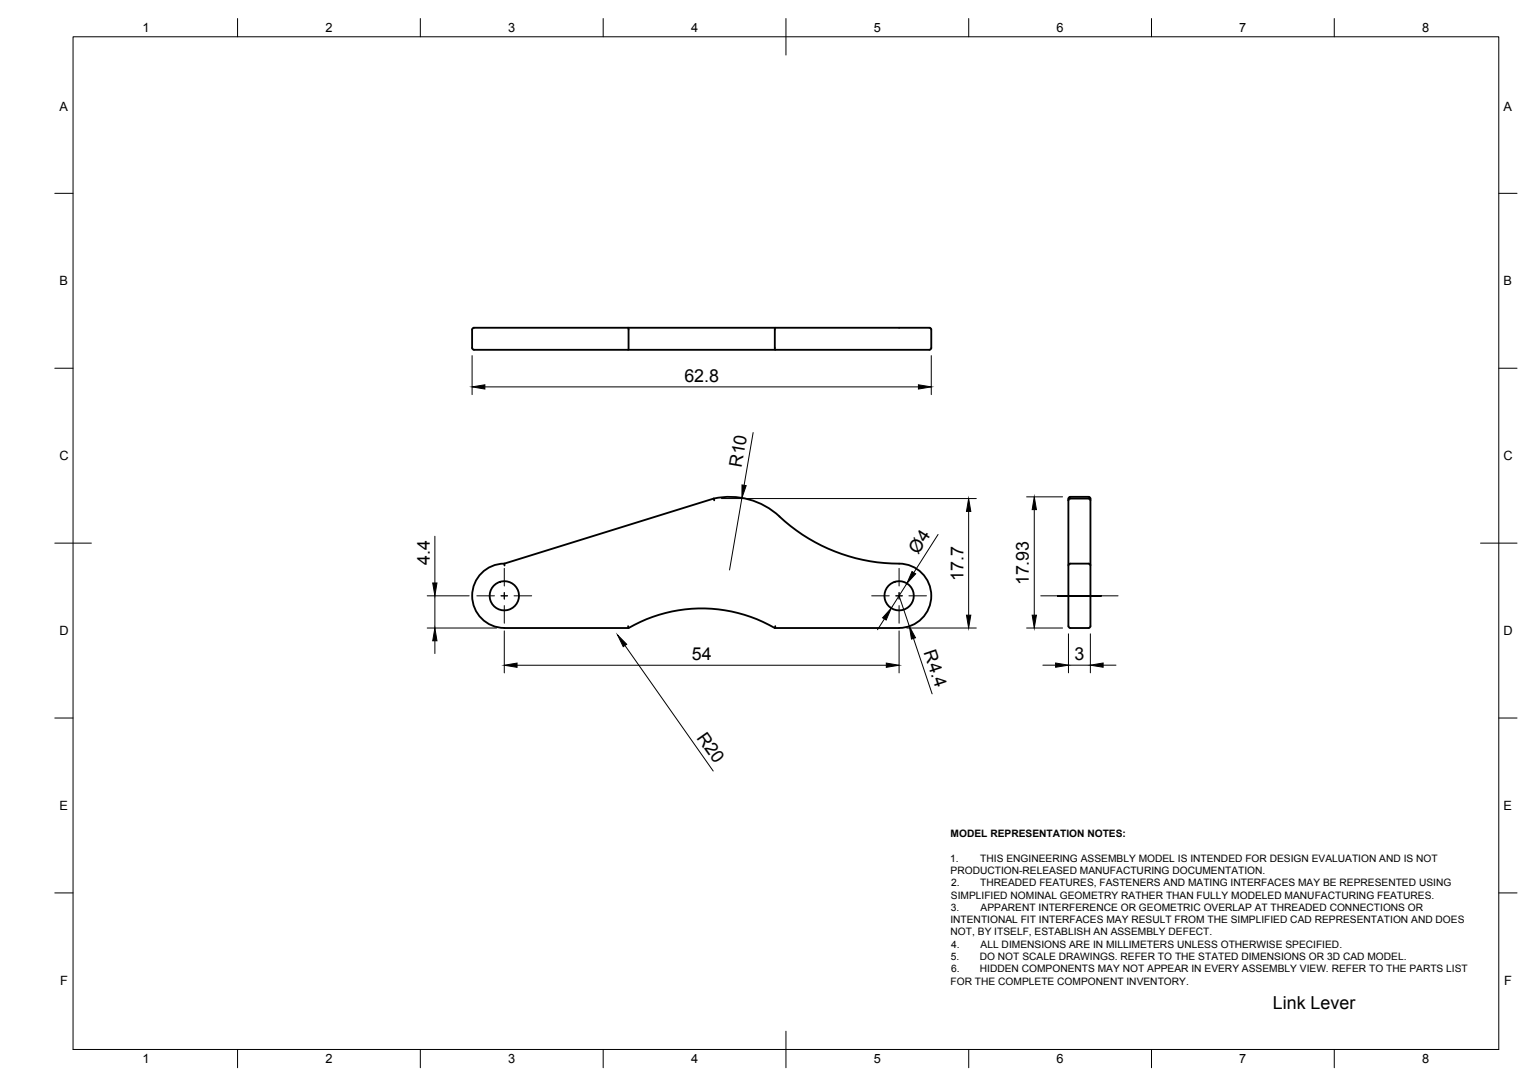
ISO-10303-21;
HEADER;
/* Generated by software containing ST-Developer
 * from STEP Tools, Inc. (www.steptools.com) 
 */

FILE_DESCRIPTION(
/* description */ ('STEP AP214'),
/* implementation_level */ '2;1');

FILE_NAME(
/* name */ 'Link Lever.step',
/* time_stamp */ '2026-10-06T11:11:25-07:00',
/* author */ (''),
/* organization */ (''),
/* preprocessor_version */ 'ST-DEVELOPER v20.2',
/* originating_system */ 'Autodesk Translation Framework v15.15.0.0',
/* authorisation */ '');

FILE_SCHEMA (('AUTOMOTIVE_DESIGN { 1 0 10303 214 3 1 1 }'));
ENDSEC;

DATA;
#10=MECHANICAL_DESIGN_GEOMETRIC_PRESENTATION_REPRESENTATION('',(#709),#47717);
#518=B_SPLINE_CURVE_WITH_KNOTS('',3,(#47531,#47532,#47533,#47534,#47535,
#47536,#47537,#47538,#47539,#47540,#47541,#47542,#47543,#47544),
 .UNSPECIFIED.,.F.,.F.,(4,2,2,2,2,2,4),(0.039886669715827,0.0401044661515991,
0.0495727843168759,0.0592161981418575,0.0692076983643014,0.0797697497054474,
0.0800012054326904),.UNSPECIFIED.);
#519=B_SPLINE_CURVE_WITH_KNOTS('',3,(#47547,#47548,#47549,#47550,#47551,
#47552,#47553,#47554,#47555,#47556,#47557,#47558),.UNSPECIFIED.,.F.,.F.,
(4,2,2,2,2,4),(-0.000230133150951674,0.,0.0101766413292995,0.0200160913840905,
0.0297402908990685,0.0394076883089345),.UNSPECIFIED.);
#520=B_SPLINE_CURVE_WITH_KNOTS('',3,(#47560,#47561,#47562,#47563,#47564,
#47565,#47566,#47567,#47568,#47569,#47570,#47571),.UNSPECIFIED.,.F.,.F.,
(4,2,2,2,2,4),(-0.0398866697156879,-0.0305471274410706,-0.0206752787312571,
-0.010434866365749,0.,0.000231445227518166),.UNSPECIFIED.);
#521=B_SPLINE_CURVE_WITH_KNOTS('',3,(#47573,#47574,#47575,#47576,#47577,
#47578,#47579,#47580,#47581,#47582,#47583,#47584,#47585,#47586,#47587,#47588,
#47589,#47590,#47591,#47592,#47593,#47594,#47595,#47596,#47597,#47598,#47599,
#47600),.UNSPECIFIED.,.F.,.F.,(4,3,3,3,3,3,3,3,3,4),(-1.09105494845026E-5,
3.84251023745443E-5,8.55160249623879E-5,0.000132661739759183,0.000179909175493616,
0.000186432057951685,0.00023702907904941,0.000287481797438324,0.000337436285325506,
0.000383774665387872),.UNSPECIFIED.);
#522=B_SPLINE_CURVE_WITH_KNOTS('',3,(#47606,#47607,#47608,#47609,#47610,
#47611,#47612,#47613,#47614,#47615,#47616,#47617),.UNSPECIFIED.,.F.,.F.,
(4,2,2,2,2,4),(-0.0790455097686946,-0.0788153766177156,-0.0686387352884633,
-0.0587992852337163,-0.0490750857187486,-0.0394076883088853),
 .UNSPECIFIED.);
#523=B_SPLINE_CURVE_WITH_KNOTS('',3,(#47618,#47619,#47620,#47621,#47622,
#47623,#47624,#47625,#47626,#47627,#47628,#47629,#47630,#47631,#47632,#47633,
#47634,#47635,#47636,#47637,#47638,#47639,#47640,#47641,#47642,#47643,#47644,
#47645),.UNSPECIFIED.,.F.,.F.,(4,3,3,3,3,3,3,3,3,4),(0.,4.94468472281981E-5,
9.92247531380756E-5,0.00014929675610942,0.000195377841020618,0.000238646755348352,
0.000281883277306065,0.00032509948720421,0.000368395674290727,0.000390755682041237),
 .UNSPECIFIED.);
#524=B_SPLINE_CURVE_WITH_KNOTS('',3,(#47652,#47653,#47654,#47655,#47656,
#47657,#47658,#47659,#47660,#47661,#47662,#47663),.UNSPECIFIED.,.F.,.F.,
(4,2,2,2,2,4),(-0.000231445227522379,0.,0.0104348663658747,0.0206752787314242,
0.0305471274412819,0.0398866697158144),.UNSPECIFIED.);
#525=B_SPLINE_CURVE_WITH_KNOTS('',3,(#47665,#47666,#47667,#47668,#47669,
#47670,#47671,#47672,#47673,#47674,#47675,#47676),.UNSPECIFIED.,.F.,.F.,
(4,2,2,2,2,4),(-0.0799975657698679,-0.0797661310415978,-0.0693317380416801,
-0.0590917902207848,-0.0492203893360867,-0.0398812707391191),
 .UNSPECIFIED.);
#660=TOROIDAL_SURFACE('',#9872,2.25,0.25);
#661=TOROIDAL_SURFACE('',#9876,4.15,0.25);
#662=TOROIDAL_SURFACE('',#9881,2.25,0.25);
#663=TOROIDAL_SURFACE('',#9885,4.15,0.25);
#664=TOROIDAL_SURFACE('',#9890,2.25,0.25);
#665=TOROIDAL_SURFACE('',#9894,2.25,0.25);
#666=TOROIDAL_SURFACE('',#9928,4.15,0.25);
#667=TOROIDAL_SURFACE('',#9929,20.25,0.25);
#668=TOROIDAL_SURFACE('',#9932,9.75,0.25);
#669=TOROIDAL_SURFACE('',#9934,24.25,0.25);
#670=TOROIDAL_SURFACE('',#9936,9.75,0.25);
#671=TOROIDAL_SURFACE('',#9938,4.15,0.25);
#672=TOROIDAL_SURFACE('',#9940,24.25,0.25);
#673=TOROIDAL_SURFACE('',#9942,20.25,0.25);
#685=SHAPE_REPRESENTATION_RELATIONSHIP('SRR','None',#47772,#697);
#697=ADVANCED_BREP_SHAPE_REPRESENTATION('',(#721),#47716);
#709=STYLED_ITEM('',(#47830),#721);
#721=MANIFOLD_SOLID_BREP('Body1',#8936);
#755=FACE_BOUND('',#3098,.T.);
#756=FACE_BOUND('',#3099,.T.);
#757=FACE_BOUND('',#3101,.T.);
#758=FACE_BOUND('',#3102,.T.);
#878=PLANE('',#9901);
#879=PLANE('',#9906);
#880=PLANE('',#9911);
#881=PLANE('',#9915);
#882=PLANE('',#9919);
#1348=LINE('',#47457,#1835);
#1349=LINE('',#47459,#1836);
#1350=LINE('',#47461,#1837);
#1351=LINE('',#47462,#1838);
#1352=LINE('',#47469,#1839);
#1353=LINE('',#47473,#1840);
#1354=LINE('',#47476,#1841);
#1355=LINE('',#47481,#1842);
#1356=LINE('',#47487,#1843);
#1357=LINE('',#47490,#1844);
#1358=LINE('',#47494,#1845);
#1359=LINE('',#47495,#1846);
#1360=LINE('',#47496,#1847);
#1361=LINE('',#47500,#1848);
#1362=LINE('',#47506,#1849);
#1363=LINE('',#47507,#1850);
#1364=LINE('',#47508,#1851);
#1365=LINE('',#47512,#1852);
#1366=LINE('',#47518,#1853);
#1367=LINE('',#47519,#1854);
#1368=LINE('',#47520,#1855);
#1369=LINE('',#47524,#1856);
#1835=VECTOR('',#12079,1.99999999999999);
#1836=VECTOR('',#12082,2.);
#1837=VECTOR('',#12085,1000.);
#1838=VECTOR('',#12086,1000.);
#1839=VECTOR('',#12093,1000.);
#1840=VECTOR('',#12096,1000.);
#1841=VECTOR('',#12099,1000.);
#1842=VECTOR('',#12104,1000.);
#1843=VECTOR('',#12109,1000.);
#1844=VECTOR('',#12112,1000.);
#1845=VECTOR('',#12115,1000.);
#1846=VECTOR('',#12116,1000.);
#1847=VECTOR('',#12117,1000.);
#1848=VECTOR('',#12120,1000.);
#1849=VECTOR('',#12127,1000.);
#1850=VECTOR('',#12128,1000.);
#1851=VECTOR('',#12129,1000.);
#1852=VECTOR('',#12132,1000.);
#1853=VECTOR('',#12139,1000.);
#1854=VECTOR('',#12140,1000.);
#1855=VECTOR('',#12141,1000.);
#1856=VECTOR('',#12144,1000.);
#2050=CYLINDRICAL_SURFACE('',#9898,1.99999999999999);
#2051=CYLINDRICAL_SURFACE('',#9899,2.);
#2052=CYLINDRICAL_SURFACE('',#9900,4.4);
#2053=CYLINDRICAL_SURFACE('',#9912,20.);
#2054=CYLINDRICAL_SURFACE('',#9916,4.4);
#2055=CYLINDRICAL_SURFACE('',#9920,9.99999999999999);
#2056=CYLINDRICAL_SURFACE('',#9923,24.);
#2057=CYLINDRICAL_SURFACE('',#9926,0.25);
#2058=CYLINDRICAL_SURFACE('',#9930,0.250000000000004);
#2059=CYLINDRICAL_SURFACE('',#9931,0.25);
#2060=CYLINDRICAL_SURFACE('',#9935,0.250000000000004);
#2061=CYLINDRICAL_SURFACE('',#9941,0.25);
#2062=CYLINDRICAL_SURFACE('',#9943,0.25);
#2543=FACE_OUTER_BOUND('',#3088,.T.);
#2544=FACE_OUTER_BOUND('',#3089,.T.);
#2545=FACE_OUTER_BOUND('',#3090,.T.);
#2546=FACE_OUTER_BOUND('',#3091,.T.);
#2547=FACE_OUTER_BOUND('',#3092,.T.);
#2548=FACE_OUTER_BOUND('',#3093,.T.);
#2549=FACE_OUTER_BOUND('',#3094,.T.);
#2550=FACE_OUTER_BOUND('',#3095,.T.);
#2551=FACE_OUTER_BOUND('',#3096,.T.);
#2552=FACE_OUTER_BOUND('',#3097,.T.);
#2553=FACE_OUTER_BOUND('',#3100,.T.);
#2554=FACE_OUTER_BOUND('',#3103,.T.);
#2555=FACE_OUTER_BOUND('',#3104,.T.);
#2556=FACE_OUTER_BOUND('',#3105,.T.);
#2557=FACE_OUTER_BOUND('',#3106,.T.);
#2558=FACE_OUTER_BOUND('',#3107,.T.);
#2559=FACE_OUTER_BOUND('',#3108,.T.);
#2560=FACE_OUTER_BOUND('',#3109,.T.);
#2561=FACE_OUTER_BOUND('',#3110,.T.);
#2562=FACE_OUTER_BOUND('',#3111,.T.);
#2563=FACE_OUTER_BOUND('',#3112,.T.);
#2564=FACE_OUTER_BOUND('',#3113,.T.);
#2565=FACE_OUTER_BOUND('',#3114,.T.);
#2566=FACE_OUTER_BOUND('',#3115,.T.);
#2567=FACE_OUTER_BOUND('',#3116,.T.);
#2568=FACE_OUTER_BOUND('',#3117,.T.);
#2569=FACE_OUTER_BOUND('',#3118,.T.);
#2570=FACE_OUTER_BOUND('',#3119,.T.);
#2571=FACE_OUTER_BOUND('',#3120,.T.);
#2572=FACE_OUTER_BOUND('',#3121,.T.);
#2573=FACE_OUTER_BOUND('',#3122,.T.);
#2574=FACE_OUTER_BOUND('',#3123,.T.);
#3088=EDGE_LOOP('',(#8263,#8264,#8265,#8266));
#3089=EDGE_LOOP('',(#8267,#8268,#8269,#8270));
#3090=EDGE_LOOP('',(#8271,#8272,#8273,#8274));
#3091=EDGE_LOOP('',(#8275,#8276,#8277,#8278));
#3092=EDGE_LOOP('',(#8279,#8280,#8281,#8282));
#3093=EDGE_LOOP('',(#8283,#8284,#8285,#8286));
#3094=EDGE_LOOP('',(#8287,#8288,#8289,#8290));
#3095=EDGE_LOOP('',(#8291,#8292,#8293,#8294));
#3096=EDGE_LOOP('',(#8295,#8296,#8297,#8298));
#3097=EDGE_LOOP('',(#8299,#8300,#8301,#8302,#8303,#8304,#8305,#8306));
#3098=EDGE_LOOP('',(#8307));
#3099=EDGE_LOOP('',(#8308));
#3100=EDGE_LOOP('',(#8309,#8310,#8311,#8312,#8313,#8314,#8315,#8316));
#3101=EDGE_LOOP('',(#8317));
#3102=EDGE_LOOP('',(#8318));
#3103=EDGE_LOOP('',(#8319,#8320,#8321,#8322));
#3104=EDGE_LOOP('',(#8323,#8324,#8325,#8326));
#3105=EDGE_LOOP('',(#8327,#8328,#8329,#8330));
#3106=EDGE_LOOP('',(#8331,#8332,#8333,#8334));
#3107=EDGE_LOOP('',(#8335,#8336,#8337,#8338));
#3108=EDGE_LOOP('',(#8339,#8340,#8341,#8342));
#3109=EDGE_LOOP('',(#8343,#8344,#8345,#8346));
#3110=EDGE_LOOP('',(#8347,#8348,#8349,#8350));
#3111=EDGE_LOOP('',(#8351,#8352,#8353,#8354));
#3112=EDGE_LOOP('',(#8355,#8356,#8357,#8358));
#3113=EDGE_LOOP('',(#8359,#8360,#8361,#8362));
#3114=EDGE_LOOP('',(#8363,#8364,#8365,#8366));
#3115=EDGE_LOOP('',(#8367,#8368,#8369,#8370));
#3116=EDGE_LOOP('',(#8371,#8372,#8373,#8374));
#3117=EDGE_LOOP('',(#8375,#8376,#8377,#8378));
#3118=EDGE_LOOP('',(#8379,#8380,#8381,#8382));
#3119=EDGE_LOOP('',(#8383,#8384,#8385,#8386));
#3120=EDGE_LOOP('',(#8387,#8388,#8389,#8390));
#3121=EDGE_LOOP('',(#8391,#8392,#8393,#8394));
#3122=EDGE_LOOP('',(#8395,#8396,#8397,#8398));
#3123=EDGE_LOOP('',(#8399,#8400,#8401,#8402));
#3492=CIRCLE('',#9873,2.);
#3493=CIRCLE('',#9874,0.25);
#3494=CIRCLE('',#9875,2.25);
#3495=CIRCLE('',#9877,4.4);
#3496=CIRCLE('',#9878,0.25);
#3497=CIRCLE('',#9879,4.15);
#3498=CIRCLE('',#9880,0.25);
#3499=CIRCLE('',#9882,1.99999999999999);
#3500=CIRCLE('',#9883,0.25);
#3501=CIRCLE('',#9884,2.24999999999999);
#3502=CIRCLE('',#9886,4.15);
#3503=CIRCLE('',#9887,0.25);
#3504=CIRCLE('',#9888,4.4);
#3505=CIRCLE('',#9889,0.25);
#3506=CIRCLE('',#9891,2.25);
#3507=CIRCLE('',#9892,0.25);
#3508=CIRCLE('',#9893,2.);
#3509=CIRCLE('',#9895,2.25);
#3510=CIRCLE('',#9896,0.25);
#3511=CIRCLE('',#9897,2.00000000000001);
#3512=CIRCLE('',#9902,9.75);
#3513=CIRCLE('',#9903,24.25);
#3514=CIRCLE('',#9904,20.25);
#3515=CIRCLE('',#9905,4.15);
#3516=CIRCLE('',#9907,20.25);
#3517=CIRCLE('',#9908,24.25);
#3518=CIRCLE('',#9909,9.74999999999999);
#3519=CIRCLE('',#9910,4.15);
#3520=CIRCLE('',#9913,20.);
#3521=CIRCLE('',#9914,20.);
#3522=CIRCLE('',#9917,4.4);
#3523=CIRCLE('',#9918,4.4);
#3524=CIRCLE('',#9921,9.99999999999999);
#3525=CIRCLE('',#9922,9.99999999999999);
#3526=CIRCLE('',#9924,24.);
#3527=CIRCLE('',#9925,24.);
#3528=CIRCLE('',#9927,0.25);
#3529=CIRCLE('',#9933,0.249999999999998);
#3530=CIRCLE('',#9937,0.249999999999998);
#3531=CIRCLE('',#9939,0.25);
#4349=VERTEX_POINT('',#47415);
#4350=VERTEX_POINT('',#47417);
#4351=VERTEX_POINT('',#47421);
#4352=VERTEX_POINT('',#47422);
#4353=VERTEX_POINT('',#47424);
#4354=VERTEX_POINT('',#47426);
#4355=VERTEX_POINT('',#47430);
#4356=VERTEX_POINT('',#47432);
#4357=VERTEX_POINT('',#47436);
#4358=VERTEX_POINT('',#47437);
#4359=VERTEX_POINT('',#47439);
#4360=VERTEX_POINT('',#47441);
#4361=VERTEX_POINT('',#47445);
#4362=VERTEX_POINT('',#47447);
#4363=VERTEX_POINT('',#47451);
#4364=VERTEX_POINT('',#47453);
#4365=VERTEX_POINT('',#47464);
#4366=VERTEX_POINT('',#47465);
#4367=VERTEX_POINT('',#47468);
#4368=VERTEX_POINT('',#47470);
#4369=VERTEX_POINT('',#47472);
#4370=VERTEX_POINT('',#47474);
#4371=VERTEX_POINT('',#47478);
#4372=VERTEX_POINT('',#47479);
#4373=VERTEX_POINT('',#47482);
#4374=VERTEX_POINT('',#47484);
#4375=VERTEX_POINT('',#47486);
#4376=VERTEX_POINT('',#47488);
#4377=VERTEX_POINT('',#47492);
#4378=VERTEX_POINT('',#47493);
#4379=VERTEX_POINT('',#47498);
#4380=VERTEX_POINT('',#47499);
#4381=VERTEX_POINT('',#47504);
#4382=VERTEX_POINT('',#47505);
#4383=VERTEX_POINT('',#47510);
#4384=VERTEX_POINT('',#47511);
#4385=VERTEX_POINT('',#47516);
#4386=VERTEX_POINT('',#47517);
#4387=VERTEX_POINT('',#47522);
#4388=VERTEX_POINT('',#47523);
#5657=EDGE_CURVE('',#4349,#4349,#3492,.T.);
#5658=EDGE_CURVE('',#4349,#4350,#3493,.T.);
#5659=EDGE_CURVE('',#4350,#4350,#3494,.T.);
#5660=EDGE_CURVE('',#4351,#4352,#3495,.T.);
#5661=EDGE_CURVE('',#4351,#4353,#3496,.T.);
#5662=EDGE_CURVE('',#4354,#4353,#3497,.T.);
#5663=EDGE_CURVE('',#4352,#4354,#3498,.T.);
#5664=EDGE_CURVE('',#4355,#4355,#3499,.T.);
#5665=EDGE_CURVE('',#4355,#4356,#3500,.T.);
#5666=EDGE_CURVE('',#4356,#4356,#3501,.T.);
#5667=EDGE_CURVE('',#4357,#4358,#3502,.T.);
#5668=EDGE_CURVE('',#4359,#4357,#3503,.T.);
#5669=EDGE_CURVE('',#4360,#4359,#3504,.T.);
#5670=EDGE_CURVE('',#4360,#4358,#3505,.T.);
#5671=EDGE_CURVE('',#4361,#4361,#3506,.T.);
#5672=EDGE_CURVE('',#4361,#4362,#3507,.T.);
#5673=EDGE_CURVE('',#4362,#4362,#3508,.T.);
#5674=EDGE_CURVE('',#4363,#4363,#3509,.T.);
#5675=EDGE_CURVE('',#4363,#4364,#3510,.T.);
#5676=EDGE_CURVE('',#4364,#4364,#3511,.T.);
#5677=EDGE_CURVE('',#4364,#4355,#1348,.T.);
#5678=EDGE_CURVE('',#4362,#4349,#1349,.T.);
#5679=EDGE_CURVE('',#4359,#4351,#1350,.T.);
#5680=EDGE_CURVE('',#4360,#4352,#1351,.T.);
#5681=EDGE_CURVE('',#4365,#4366,#3512,.T.);
#5682=EDGE_CURVE('',#4366,#4357,#3513,.T.);
#5683=EDGE_CURVE('',#4358,#4367,#1352,.T.);
#5684=EDGE_CURVE('',#4367,#4368,#3514,.T.);
#5685=EDGE_CURVE('',#4368,#4369,#1353,.T.);
#5686=EDGE_CURVE('',#4369,#4370,#3515,.T.);
#5687=EDGE_CURVE('',#4370,#4365,#1354,.T.);
#5688=EDGE_CURVE('',#4371,#4372,#3516,.T.);
#5689=EDGE_CURVE('',#4372,#4354,#1355,.T.);
#5690=EDGE_CURVE('',#4353,#4373,#3517,.T.);
#5691=EDGE_CURVE('',#4373,#4374,#3518,.T.);
#5692=EDGE_CURVE('',#4374,#4375,#1356,.T.);
#5693=EDGE_CURVE('',#4375,#4376,#3519,.T.);
#5694=EDGE_CURVE('',#4376,#4371,#1357,.T.);
#5695=EDGE_CURVE('',#4377,#4378,#1358,.T.);
#5696=EDGE_CURVE('',#4377,#4360,#1359,.T.);
#5697=EDGE_CURVE('',#4352,#4378,#1360,.T.);
#5698=EDGE_CURVE('',#4379,#4380,#1361,.T.);
#5699=EDGE_CURVE('',#4379,#4377,#3520,.T.);
#5700=EDGE_CURVE('',#4378,#4380,#3521,.T.);
#5701=EDGE_CURVE('',#4381,#4382,#1362,.T.);
#5702=EDGE_CURVE('',#4381,#4379,#1363,.T.);
#5703=EDGE_CURVE('',#4380,#4382,#1364,.T.);
#5704=EDGE_CURVE('',#4383,#4384,#1365,.T.);
#5705=EDGE_CURVE('',#4383,#4381,#3522,.T.);
#5706=EDGE_CURVE('',#4382,#4384,#3523,.T.);
#5707=EDGE_CURVE('',#4385,#4386,#1366,.T.);
#5708=EDGE_CURVE('',#4385,#4383,#1367,.T.);
#5709=EDGE_CURVE('',#4384,#4386,#1368,.T.);
#5710=EDGE_CURVE('',#4387,#4388,#1369,.T.);
#5711=EDGE_CURVE('',#4387,#4385,#3524,.T.);
#5712=EDGE_CURVE('',#4386,#4388,#3525,.T.);
#5713=EDGE_CURVE('',#4359,#4387,#3526,.T.);
#5714=EDGE_CURVE('',#4388,#4351,#3527,.T.);
#5715=EDGE_CURVE('',#4379,#4368,#518,.T.);
#5716=EDGE_CURVE('',#4369,#4381,#3528,.T.);
#5717=EDGE_CURVE('',#4370,#4383,#519,.T.);
#5718=EDGE_CURVE('',#4377,#4367,#520,.T.);
#5719=EDGE_CURVE('',#4365,#4385,#521,.T.);
#5720=EDGE_CURVE('',#4366,#4387,#3529,.T.);
#5721=EDGE_CURVE('',#4375,#4384,#522,.T.);
#5722=EDGE_CURVE('',#4386,#4374,#523,.T.);
#5723=EDGE_CURVE('',#4388,#4373,#3530,.T.);
#5724=EDGE_CURVE('',#4376,#4382,#3531,.T.);
#5725=EDGE_CURVE('',#4371,#4380,#524,.T.);
#5726=EDGE_CURVE('',#4372,#4378,#525,.T.);
#8263=ORIENTED_EDGE('',*,*,#5657,.F.);
#8264=ORIENTED_EDGE('',*,*,#5658,.T.);
#8265=ORIENTED_EDGE('',*,*,#5659,.F.);
#8266=ORIENTED_EDGE('',*,*,#5658,.F.);
#8267=ORIENTED_EDGE('',*,*,#5660,.F.);
#8268=ORIENTED_EDGE('',*,*,#5661,.T.);
#8269=ORIENTED_EDGE('',*,*,#5662,.F.);
#8270=ORIENTED_EDGE('',*,*,#5663,.F.);
#8271=ORIENTED_EDGE('',*,*,#5664,.F.);
#8272=ORIENTED_EDGE('',*,*,#5665,.T.);
#8273=ORIENTED_EDGE('',*,*,#5666,.F.);
#8274=ORIENTED_EDGE('',*,*,#5665,.F.);
#8275=ORIENTED_EDGE('',*,*,#5667,.F.);
#8276=ORIENTED_EDGE('',*,*,#5668,.F.);
#8277=ORIENTED_EDGE('',*,*,#5669,.F.);
#8278=ORIENTED_EDGE('',*,*,#5670,.T.);
#8279=ORIENTED_EDGE('',*,*,#5671,.F.);
#8280=ORIENTED_EDGE('',*,*,#5672,.T.);
#8281=ORIENTED_EDGE('',*,*,#5673,.F.);
#8282=ORIENTED_EDGE('',*,*,#5672,.F.);
#8283=ORIENTED_EDGE('',*,*,#5674,.F.);
#8284=ORIENTED_EDGE('',*,*,#5675,.T.);
#8285=ORIENTED_EDGE('',*,*,#5676,.F.);
#8286=ORIENTED_EDGE('',*,*,#5675,.F.);
#8287=ORIENTED_EDGE('',*,*,#5676,.T.);
#8288=ORIENTED_EDGE('',*,*,#5677,.T.);
#8289=ORIENTED_EDGE('',*,*,#5664,.T.);
#8290=ORIENTED_EDGE('',*,*,#5677,.F.);
#8291=ORIENTED_EDGE('',*,*,#5673,.T.);
#8292=ORIENTED_EDGE('',*,*,#5678,.T.);
#8293=ORIENTED_EDGE('',*,*,#5657,.T.);
#8294=ORIENTED_EDGE('',*,*,#5678,.F.);
#8295=ORIENTED_EDGE('',*,*,#5669,.T.);
#8296=ORIENTED_EDGE('',*,*,#5679,.T.);
#8297=ORIENTED_EDGE('',*,*,#5660,.T.);
#8298=ORIENTED_EDGE('',*,*,#5680,.F.);
#8299=ORIENTED_EDGE('',*,*,#5681,.T.);
#8300=ORIENTED_EDGE('',*,*,#5682,.T.);
#8301=ORIENTED_EDGE('',*,*,#5667,.T.);
#8302=ORIENTED_EDGE('',*,*,#5683,.T.);
#8303=ORIENTED_EDGE('',*,*,#5684,.T.);
#8304=ORIENTED_EDGE('',*,*,#5685,.T.);
#8305=ORIENTED_EDGE('',*,*,#5686,.T.);
#8306=ORIENTED_EDGE('',*,*,#5687,.T.);
#8307=ORIENTED_EDGE('',*,*,#5674,.T.);
#8308=ORIENTED_EDGE('',*,*,#5671,.T.);
#8309=ORIENTED_EDGE('',*,*,#5688,.T.);
#8310=ORIENTED_EDGE('',*,*,#5689,.T.);
#8311=ORIENTED_EDGE('',*,*,#5662,.T.);
#8312=ORIENTED_EDGE('',*,*,#5690,.T.);
#8313=ORIENTED_EDGE('',*,*,#5691,.T.);
#8314=ORIENTED_EDGE('',*,*,#5692,.T.);
#8315=ORIENTED_EDGE('',*,*,#5693,.T.);
#8316=ORIENTED_EDGE('',*,*,#5694,.T.);
#8317=ORIENTED_EDGE('',*,*,#5659,.T.);
#8318=ORIENTED_EDGE('',*,*,#5666,.T.);
#8319=ORIENTED_EDGE('',*,*,#5695,.F.);
#8320=ORIENTED_EDGE('',*,*,#5696,.T.);
#8321=ORIENTED_EDGE('',*,*,#5680,.T.);
#8322=ORIENTED_EDGE('',*,*,#5697,.T.);
#8323=ORIENTED_EDGE('',*,*,#5698,.F.);
#8324=ORIENTED_EDGE('',*,*,#5699,.T.);
#8325=ORIENTED_EDGE('',*,*,#5695,.T.);
#8326=ORIENTED_EDGE('',*,*,#5700,.T.);
#8327=ORIENTED_EDGE('',*,*,#5701,.F.);
#8328=ORIENTED_EDGE('',*,*,#5702,.T.);
#8329=ORIENTED_EDGE('',*,*,#5698,.T.);
#8330=ORIENTED_EDGE('',*,*,#5703,.T.);
#8331=ORIENTED_EDGE('',*,*,#5704,.F.);
#8332=ORIENTED_EDGE('',*,*,#5705,.T.);
#8333=ORIENTED_EDGE('',*,*,#5701,.T.);
#8334=ORIENTED_EDGE('',*,*,#5706,.T.);
#8335=ORIENTED_EDGE('',*,*,#5707,.F.);
#8336=ORIENTED_EDGE('',*,*,#5708,.T.);
#8337=ORIENTED_EDGE('',*,*,#5704,.T.);
#8338=ORIENTED_EDGE('',*,*,#5709,.T.);
#8339=ORIENTED_EDGE('',*,*,#5710,.F.);
#8340=ORIENTED_EDGE('',*,*,#5711,.T.);
#8341=ORIENTED_EDGE('',*,*,#5707,.T.);
#8342=ORIENTED_EDGE('',*,*,#5712,.T.);
#8343=ORIENTED_EDGE('',*,*,#5679,.F.);
#8344=ORIENTED_EDGE('',*,*,#5713,.T.);
#8345=ORIENTED_EDGE('',*,*,#5710,.T.);
#8346=ORIENTED_EDGE('',*,*,#5714,.T.);
#8347=ORIENTED_EDGE('',*,*,#5715,.F.);
#8348=ORIENTED_EDGE('',*,*,#5702,.F.);
#8349=ORIENTED_EDGE('',*,*,#5716,.F.);
#8350=ORIENTED_EDGE('',*,*,#5685,.F.);
#8351=ORIENTED_EDGE('',*,*,#5716,.T.);
#8352=ORIENTED_EDGE('',*,*,#5705,.F.);
#8353=ORIENTED_EDGE('',*,*,#5717,.F.);
#8354=ORIENTED_EDGE('',*,*,#5686,.F.);
#8355=ORIENTED_EDGE('',*,*,#5715,.T.);
#8356=ORIENTED_EDGE('',*,*,#5684,.F.);
#8357=ORIENTED_EDGE('',*,*,#5718,.F.);
#8358=ORIENTED_EDGE('',*,*,#5699,.F.);
#8359=ORIENTED_EDGE('',*,*,#5717,.T.);
#8360=ORIENTED_EDGE('',*,*,#5708,.F.);
#8361=ORIENTED_EDGE('',*,*,#5719,.F.);
#8362=ORIENTED_EDGE('',*,*,#5687,.F.);
#8363=ORIENTED_EDGE('',*,*,#5718,.T.);
#8364=ORIENTED_EDGE('',*,*,#5683,.F.);
#8365=ORIENTED_EDGE('',*,*,#5670,.F.);
#8366=ORIENTED_EDGE('',*,*,#5696,.F.);
#8367=ORIENTED_EDGE('',*,*,#5719,.T.);
#8368=ORIENTED_EDGE('',*,*,#5711,.F.);
#8369=ORIENTED_EDGE('',*,*,#5720,.F.);
#8370=ORIENTED_EDGE('',*,*,#5681,.F.);
#8371=ORIENTED_EDGE('',*,*,#5720,.T.);
#8372=ORIENTED_EDGE('',*,*,#5713,.F.);
#8373=ORIENTED_EDGE('',*,*,#5668,.T.);
#8374=ORIENTED_EDGE('',*,*,#5682,.F.);
#8375=ORIENTED_EDGE('',*,*,#5721,.F.);
#8376=ORIENTED_EDGE('',*,*,#5692,.F.);
#8377=ORIENTED_EDGE('',*,*,#5722,.F.);
#8378=ORIENTED_EDGE('',*,*,#5709,.F.);
#8379=ORIENTED_EDGE('',*,*,#5722,.T.);
#8380=ORIENTED_EDGE('',*,*,#5691,.F.);
#8381=ORIENTED_EDGE('',*,*,#5723,.F.);
#8382=ORIENTED_EDGE('',*,*,#5712,.F.);
#8383=ORIENTED_EDGE('',*,*,#5721,.T.);
#8384=ORIENTED_EDGE('',*,*,#5706,.F.);
#8385=ORIENTED_EDGE('',*,*,#5724,.F.);
#8386=ORIENTED_EDGE('',*,*,#5693,.F.);
#8387=ORIENTED_EDGE('',*,*,#5723,.T.);
#8388=ORIENTED_EDGE('',*,*,#5690,.F.);
#8389=ORIENTED_EDGE('',*,*,#5661,.F.);
#8390=ORIENTED_EDGE('',*,*,#5714,.F.);
#8391=ORIENTED_EDGE('',*,*,#5724,.T.);
#8392=ORIENTED_EDGE('',*,*,#5703,.F.);
#8393=ORIENTED_EDGE('',*,*,#5725,.F.);
#8394=ORIENTED_EDGE('',*,*,#5694,.F.);
#8395=ORIENTED_EDGE('',*,*,#5725,.T.);
#8396=ORIENTED_EDGE('',*,*,#5700,.F.);
#8397=ORIENTED_EDGE('',*,*,#5726,.F.);
#8398=ORIENTED_EDGE('',*,*,#5688,.F.);
#8399=ORIENTED_EDGE('',*,*,#5663,.T.);
#8400=ORIENTED_EDGE('',*,*,#5689,.F.);
#8401=ORIENTED_EDGE('',*,*,#5726,.T.);
#8402=ORIENTED_EDGE('',*,*,#5697,.F.);
#8893=ADVANCED_FACE('',(#2543),#660,.T.);
#8894=ADVANCED_FACE('',(#2544),#661,.T.);
#8895=ADVANCED_FACE('',(#2545),#662,.T.);
#8896=ADVANCED_FACE('',(#2546),#663,.T.);
#8897=ADVANCED_FACE('',(#2547),#664,.T.);
#8898=ADVANCED_FACE('',(#2548),#665,.T.);
#8899=ADVANCED_FACE('',(#2549),#2050,.F.);
#8900=ADVANCED_FACE('',(#2550),#2051,.F.);
#8901=ADVANCED_FACE('',(#2551),#2052,.T.);
#8902=ADVANCED_FACE('',(#2552,#755,#756),#878,.F.);
#8903=ADVANCED_FACE('',(#2553,#757,#758),#879,.T.);
#8904=ADVANCED_FACE('',(#2554),#880,.F.);
#8905=ADVANCED_FACE('',(#2555),#2053,.F.);
#8906=ADVANCED_FACE('',(#2556),#881,.F.);
#8907=ADVANCED_FACE('',(#2557),#2054,.T.);
#8908=ADVANCED_FACE('',(#2558),#882,.F.);
#8909=ADVANCED_FACE('',(#2559),#2055,.T.);
#8910=ADVANCED_FACE('',(#2560),#2056,.F.);
#8911=ADVANCED_FACE('',(#2561),#2057,.T.);
#8912=ADVANCED_FACE('',(#2562),#666,.T.);
#8913=ADVANCED_FACE('',(#2563),#667,.T.);
#8914=ADVANCED_FACE('',(#2564),#2058,.T.);
#8915=ADVANCED_FACE('',(#2565),#2059,.T.);
#8916=ADVANCED_FACE('',(#2566),#668,.T.);
#8917=ADVANCED_FACE('',(#2567),#669,.T.);
#8918=ADVANCED_FACE('',(#2568),#2060,.T.);
#8919=ADVANCED_FACE('',(#2569),#670,.T.);
#8920=ADVANCED_FACE('',(#2570),#671,.T.);
#8921=ADVANCED_FACE('',(#2571),#672,.T.);
#8922=ADVANCED_FACE('',(#2572),#2061,.T.);
#8923=ADVANCED_FACE('',(#2573),#673,.T.);
#8924=ADVANCED_FACE('',(#2574),#2062,.T.);
#8936=CLOSED_SHELL('',(#8893,#8894,#8895,#8896,#8897,#8898,#8899,#8900,
#8901,#8902,#8903,#8904,#8905,#8906,#8907,#8908,#8909,#8910,#8911,#8912,
#8913,#8914,#8915,#8916,#8917,#8918,#8919,#8920,#8921,#8922,#8923,#8924));
#9871=AXIS2_PLACEMENT_3D('',#47413,#12023,#12024);
#9872=AXIS2_PLACEMENT_3D('',#47414,#12025,#12026);
#9873=AXIS2_PLACEMENT_3D('',#47416,#12027,#12028);
#9874=AXIS2_PLACEMENT_3D('',#47418,#12029,#12030);
#9875=AXIS2_PLACEMENT_3D('',#47419,#12031,#12032);
#9876=AXIS2_PLACEMENT_3D('',#47420,#12033,#12034);
#9877=AXIS2_PLACEMENT_3D('',#47423,#12035,#12036);
#9878=AXIS2_PLACEMENT_3D('',#47425,#12037,#12038);
#9879=AXIS2_PLACEMENT_3D('',#47427,#12039,#12040);
#9880=AXIS2_PLACEMENT_3D('',#47428,#12041,#12042);
#9881=AXIS2_PLACEMENT_3D('',#47429,#12043,#12044);
#9882=AXIS2_PLACEMENT_3D('',#47431,#12045,#12046);
#9883=AXIS2_PLACEMENT_3D('',#47433,#12047,#12048);
#9884=AXIS2_PLACEMENT_3D('',#47434,#12049,#12050);
#9885=AXIS2_PLACEMENT_3D('',#47435,#12051,#12052);
#9886=AXIS2_PLACEMENT_3D('',#47438,#12053,#12054);
#9887=AXIS2_PLACEMENT_3D('',#47440,#12055,#12056);
#9888=AXIS2_PLACEMENT_3D('',#47442,#12057,#12058);
#9889=AXIS2_PLACEMENT_3D('',#47443,#12059,#12060);
#9890=AXIS2_PLACEMENT_3D('',#47444,#12061,#12062);
#9891=AXIS2_PLACEMENT_3D('',#47446,#12063,#12064);
#9892=AXIS2_PLACEMENT_3D('',#47448,#12065,#12066);
#9893=AXIS2_PLACEMENT_3D('',#47449,#12067,#12068);
#9894=AXIS2_PLACEMENT_3D('',#47450,#12069,#12070);
#9895=AXIS2_PLACEMENT_3D('',#47452,#12071,#12072);
#9896=AXIS2_PLACEMENT_3D('',#47454,#12073,#12074);
#9897=AXIS2_PLACEMENT_3D('',#47455,#12075,#12076);
#9898=AXIS2_PLACEMENT_3D('',#47456,#12077,#12078);
#9899=AXIS2_PLACEMENT_3D('',#47458,#12080,#12081);
#9900=AXIS2_PLACEMENT_3D('',#47460,#12083,#12084);
#9901=AXIS2_PLACEMENT_3D('',#47463,#12087,#12088);
#9902=AXIS2_PLACEMENT_3D('',#47466,#12089,#12090);
#9903=AXIS2_PLACEMENT_3D('',#47467,#12091,#12092);
#9904=AXIS2_PLACEMENT_3D('',#47471,#12094,#12095);
#9905=AXIS2_PLACEMENT_3D('',#47475,#12097,#12098);
#9906=AXIS2_PLACEMENT_3D('',#47477,#12100,#12101);
#9907=AXIS2_PLACEMENT_3D('',#47480,#12102,#12103);
#9908=AXIS2_PLACEMENT_3D('',#47483,#12105,#12106);
#9909=AXIS2_PLACEMENT_3D('',#47485,#12107,#12108);
#9910=AXIS2_PLACEMENT_3D('',#47489,#12110,#12111);
#9911=AXIS2_PLACEMENT_3D('',#47491,#12113,#12114);
#9912=AXIS2_PLACEMENT_3D('',#47497,#12118,#12119);
#9913=AXIS2_PLACEMENT_3D('',#47501,#12121,#12122);
#9914=AXIS2_PLACEMENT_3D('',#47502,#12123,#12124);
#9915=AXIS2_PLACEMENT_3D('',#47503,#12125,#12126);
#9916=AXIS2_PLACEMENT_3D('',#47509,#12130,#12131);
#9917=AXIS2_PLACEMENT_3D('',#47513,#12133,#12134);
#9918=AXIS2_PLACEMENT_3D('',#47514,#12135,#12136);
#9919=AXIS2_PLACEMENT_3D('',#47515,#12137,#12138);
#9920=AXIS2_PLACEMENT_3D('',#47521,#12142,#12143);
#9921=AXIS2_PLACEMENT_3D('',#47525,#12145,#12146);
#9922=AXIS2_PLACEMENT_3D('',#47526,#12147,#12148);
#9923=AXIS2_PLACEMENT_3D('',#47527,#12149,#12150);
#9924=AXIS2_PLACEMENT_3D('',#47528,#12151,#12152);
#9925=AXIS2_PLACEMENT_3D('',#47529,#12153,#12154);
#9926=AXIS2_PLACEMENT_3D('',#47530,#12155,#12156);
#9927=AXIS2_PLACEMENT_3D('',#47545,#12157,#12158);
#9928=AXIS2_PLACEMENT_3D('',#47546,#12159,#12160);
#9929=AXIS2_PLACEMENT_3D('',#47559,#12161,#12162);
#9930=AXIS2_PLACEMENT_3D('',#47572,#12163,#12164);
#9931=AXIS2_PLACEMENT_3D('',#47601,#12165,#12166);
#9932=AXIS2_PLACEMENT_3D('',#47602,#12167,#12168);
#9933=AXIS2_PLACEMENT_3D('',#47603,#12169,#12170);
#9934=AXIS2_PLACEMENT_3D('',#47604,#12171,#12172);
#9935=AXIS2_PLACEMENT_3D('',#47605,#12173,#12174);
#9936=AXIS2_PLACEMENT_3D('',#47646,#12175,#12176);
#9937=AXIS2_PLACEMENT_3D('',#47647,#12177,#12178);
#9938=AXIS2_PLACEMENT_3D('',#47648,#12179,#12180);
#9939=AXIS2_PLACEMENT_3D('',#47649,#12181,#12182);
#9940=AXIS2_PLACEMENT_3D('',#47650,#12183,#12184);
#9941=AXIS2_PLACEMENT_3D('',#47651,#12185,#12186);
#9942=AXIS2_PLACEMENT_3D('',#47664,#12187,#12188);
#9943=AXIS2_PLACEMENT_3D('',#47677,#12189,#12190);
#12023=DIRECTION('axis',(0.,0.,1.));
#12024=DIRECTION('refdir',(1.,0.,0.));
#12025=DIRECTION('center_axis',(1.69724645484627E-17,2.39104395366563E-16,
-1.));
#12026=DIRECTION('ref_axis',(0.306109702391973,-0.951996244793801,0.));
#12027=DIRECTION('center_axis',(1.69724645484627E-17,2.39104395366563E-16,
-1.));
#12028=DIRECTION('ref_axis',(0.306109702391977,-0.951996244793799,-2.22431050430871E-16));
#12029=DIRECTION('center_axis',(0.9519962447938,0.306109702391975,8.9349897821304E-17));
#12030=DIRECTION('ref_axis',(-0.306109702391975,0.9519962447938,0.));
#12031=DIRECTION('center_axis',(-1.69724645484627E-17,-2.39104395366563E-16,
1.));
#12032=DIRECTION('ref_axis',(0.306109702391977,-0.951996244793799,-2.22431050430871E-16));
#12033=DIRECTION('center_axis',(1.69724645484627E-17,2.39104395366563E-16,
-1.));
#12034=DIRECTION('ref_axis',(0.306109702391976,-0.9519962447938,0.));
#12035=DIRECTION('center_axis',(-1.69724645484627E-17,-2.39104395366563E-16,
1.));
#12036=DIRECTION('ref_axis',(0.306109702391976,-0.9519962447938,-2.22431050430871E-16));
#12037=DIRECTION('center_axis',(0.306109702391976,-0.9519962447938,-2.22431050430871E-16));
#12038=DIRECTION('ref_axis',(6.80883026501286E-17,-2.1175352473573E-16,
1.));
#12039=DIRECTION('center_axis',(1.69724645484627E-17,2.39104395366563E-16,
-1.));
#12040=DIRECTION('ref_axis',(0.306109702391976,-0.9519962447938,-2.22431050430871E-16));
#12041=DIRECTION('center_axis',(-0.306109702391976,0.9519962447938,2.22431050430871E-16));
#12042=DIRECTION('ref_axis',(-6.80883026501286E-17,2.1175352473573E-16,
-1.));
#12043=DIRECTION('center_axis',(1.69724645484627E-17,2.39104395366563E-16,
-1.));
#12044=DIRECTION('ref_axis',(0.306109702391978,-0.951996244793799,0.));
#12045=DIRECTION('center_axis',(1.69724645484627E-17,2.39104395366563E-16,
-1.));
#12046=DIRECTION('ref_axis',(0.306109702391978,-0.951996244793799,-2.22431050430871E-16));
#12047=DIRECTION('center_axis',(0.951996244793799,0.306109702391978,8.93498978213047E-17));
#12048=DIRECTION('ref_axis',(-0.306109702391978,0.951996244793799,0.));
#12049=DIRECTION('center_axis',(-1.69724645484627E-17,-2.39104395366563E-16,
1.));
#12050=DIRECTION('ref_axis',(0.306109702391974,-0.9519962447938,-2.22431050430872E-16));
#12051=DIRECTION('center_axis',(1.69724645484627E-17,2.39104395366563E-16,
-1.));
#12052=DIRECTION('ref_axis',(0.306109702391976,-0.9519962447938,0.));
#12053=DIRECTION('center_axis',(-1.69724645484627E-17,-2.39104395366563E-16,
1.));
#12054=DIRECTION('ref_axis',(0.306109702391976,-0.9519962447938,-2.22431050430871E-16));
#12055=DIRECTION('center_axis',(-0.306109702391976,0.9519962447938,2.22431050430871E-16));
#12056=DIRECTION('ref_axis',(-6.80883026501286E-17,2.1175352473573E-16,
-1.));
#12057=DIRECTION('center_axis',(1.69724645484627E-17,2.39104395366563E-16,
-1.));
#12058=DIRECTION('ref_axis',(0.306109702391976,-0.9519962447938,-2.22431050430871E-16));
#12059=DIRECTION('center_axis',(0.306109702391976,-0.9519962447938,-2.22431050430871E-16));
#12060=DIRECTION('ref_axis',(6.80883026501286E-17,-2.1175352473573E-16,
1.));
#12061=DIRECTION('center_axis',(1.69724645484627E-17,2.39104395366563E-16,
-1.));
#12062=DIRECTION('ref_axis',(0.306109702391973,-0.951996244793801,0.));
#12063=DIRECTION('center_axis',(1.69724645484627E-17,2.39104395366563E-16,
-1.));
#12064=DIRECTION('ref_axis',(0.306109702391977,-0.951996244793799,-2.22431050430871E-16));
#12065=DIRECTION('center_axis',(0.9519962447938,0.306109702391975,8.9349897821304E-17));
#12066=DIRECTION('ref_axis',(-0.306109702391975,0.9519962447938,0.));
#12067=DIRECTION('center_axis',(-1.69724645484627E-17,-2.39104395366563E-16,
1.));
#12068=DIRECTION('ref_axis',(0.306109702391977,-0.951996244793799,-2.22431050430871E-16));
#12069=DIRECTION('center_axis',(1.69724645484627E-17,2.39104395366563E-16,
-1.));
#12070=DIRECTION('ref_axis',(0.306109702391978,-0.951996244793799,0.));
#12071=DIRECTION('center_axis',(1.69724645484627E-17,2.39104395366563E-16,
-1.));
#12072=DIRECTION('ref_axis',(0.306109702391977,-0.951996244793799,-2.22431050430871E-16));
#12073=DIRECTION('center_axis',(0.951996244793799,0.306109702391978,8.93498978213047E-17));
#12074=DIRECTION('ref_axis',(-0.306109702391978,0.951996244793799,0.));
#12075=DIRECTION('center_axis',(-1.69724645484627E-17,-2.39104395366563E-16,
1.));
#12076=DIRECTION('ref_axis',(0.306109702391972,-0.951996244793801,-2.22431050430872E-16));
#12077=DIRECTION('center_axis',(1.69724645484627E-17,2.39104395366563E-16,
-1.));
#12078=DIRECTION('ref_axis',(0.306109702391978,-0.951996244793799,-2.22431050430871E-16));
#12079=DIRECTION('',(1.69724645484627E-17,2.39104395366563E-16,-1.));
#12080=DIRECTION('center_axis',(1.69724645484627E-17,2.39104395366563E-16,
-1.));
#12081=DIRECTION('ref_axis',(0.306109702391977,-0.951996244793799,-2.22431050430871E-16));
#12082=DIRECTION('',(1.69724645484627E-17,2.39104395366563E-16,-1.));
#12083=DIRECTION('center_axis',(1.69724645484627E-17,2.39104395366563E-16,
-1.));
#12084=DIRECTION('ref_axis',(0.306109702391976,-0.9519962447938,-2.22431050430871E-16));
#12085=DIRECTION('',(1.69724645484627E-17,2.39104395366563E-16,-1.));
#12086=DIRECTION('',(1.69724645484627E-17,2.39104395366563E-16,-1.));
#12087=DIRECTION('center_axis',(1.69724645484627E-17,2.39104395366563E-16,
-1.));
#12088=DIRECTION('ref_axis',(0.306109702391976,-0.9519962447938,-2.22431050430872E-16));
#12089=DIRECTION('center_axis',(-1.69724645484627E-17,-2.39104395366563E-16,
1.));
#12090=DIRECTION('ref_axis',(0.306109702391974,-0.9519962447938,-2.22431050430872E-16));
#12091=DIRECTION('center_axis',(1.69724645484627E-17,2.39104395366563E-16,
-1.));
#12092=DIRECTION('ref_axis',(0.306109702391976,-0.9519962447938,-2.22431050430871E-16));
#12093=DIRECTION('',(-0.306109702391976,0.9519962447938,2.22431050430871E-16));
#12094=DIRECTION('center_axis',(1.69724645484627E-17,2.39104395366563E-16,
-1.));
#12095=DIRECTION('ref_axis',(0.306109702391976,-0.9519962447938,-2.22431050430871E-16));
#12096=DIRECTION('',(-0.306109702391976,0.9519962447938,2.22431050430871E-16));
#12097=DIRECTION('center_axis',(-1.69724645484627E-17,-2.39104395366563E-16,
1.));
#12098=DIRECTION('ref_axis',(0.306109702391974,-0.9519962447938,-2.22431050430872E-16));
#12099=DIRECTION('',(0.010034405174207,-0.999949654089045,-2.3892204885188E-16));
#12100=DIRECTION('center_axis',(1.69724645484627E-17,2.39104395366563E-16,
-1.));
#12101=DIRECTION('ref_axis',(0.306109702391976,-0.9519962447938,-2.22431050430872E-16));
#12102=DIRECTION('center_axis',(-1.69724645484627E-17,-2.39104395366563E-16,
1.));
#12103=DIRECTION('ref_axis',(0.306109702391978,-0.951996244793799,-2.22431050430871E-16));
#12104=DIRECTION('',(0.306109702391976,-0.9519962447938,-2.22431050430871E-16));
#12105=DIRECTION('center_axis',(-1.69724645484627E-17,-2.39104395366563E-16,
1.));
#12106=DIRECTION('ref_axis',(0.306109702391976,-0.9519962447938,-2.22431050430871E-16));
#12107=DIRECTION('center_axis',(1.69724645484627E-17,2.39104395366563E-16,
-1.));
#12108=DIRECTION('ref_axis',(0.306109702391976,-0.9519962447938,-2.22431050430872E-16));
#12109=DIRECTION('',(-0.010034405174207,0.999949654089045,2.3892204885188E-16));
#12110=DIRECTION('center_axis',(1.69724645484627E-17,2.39104395366563E-16,
-1.));
#12111=DIRECTION('ref_axis',(0.306109702391974,-0.9519962447938,-2.22431050430872E-16));
#12112=DIRECTION('',(0.306109702391976,-0.9519962447938,-2.22431050430871E-16));
#12113=DIRECTION('center_axis',(-0.9519962447938,-0.306109702391976,-8.93498978213041E-17));
#12114=DIRECTION('ref_axis',(-1.69724645484627E-17,-2.39104395366563E-16,
1.));
#12115=DIRECTION('',(1.69724645484627E-17,2.39104395366563E-16,-1.));
#12116=DIRECTION('',(0.306109702391976,-0.9519962447938,-2.22431050430871E-16));
#12117=DIRECTION('',(-0.306109702391976,0.9519962447938,2.22431050430871E-16));
#12118=DIRECTION('center_axis',(1.69724645484627E-17,2.39104395366563E-16,
-1.));
#12119=DIRECTION('ref_axis',(0.306109702391976,-0.9519962447938,-2.22431050430871E-16));
#12120=DIRECTION('',(1.69724645484627E-17,2.39104395366563E-16,-1.));
#12121=DIRECTION('center_axis',(-1.69724645484627E-17,-2.39104395366563E-16,
1.));
#12122=DIRECTION('ref_axis',(0.306109702391974,-0.9519962447938,-2.22431050430872E-16));
#12123=DIRECTION('center_axis',(1.69724645484627E-17,2.39104395366563E-16,
-1.));
#12124=DIRECTION('ref_axis',(0.306109702391976,-0.9519962447938,-2.22431050430871E-16));
#12125=DIRECTION('center_axis',(-0.9519962447938,-0.306109702391976,-8.93498978213041E-17));
#12126=DIRECTION('ref_axis',(-1.69724645484627E-17,-2.39104395366563E-16,
1.));
#12127=DIRECTION('',(1.69724645484627E-17,2.39104395366563E-16,-1.));
#12128=DIRECTION('',(0.306109702391976,-0.9519962447938,-2.22431050430871E-16));
#12129=DIRECTION('',(-0.306109702391976,0.9519962447938,2.22431050430871E-16));
#12130=DIRECTION('center_axis',(1.69724645484627E-17,2.39104395366563E-16,
-1.));
#12131=DIRECTION('ref_axis',(-0.306109702391977,0.951996244793799,2.22431050430871E-16));
#12132=DIRECTION('',(1.69724645484627E-17,2.39104395366563E-16,-1.));
#12133=DIRECTION('center_axis',(1.69724645484627E-17,2.39104395366563E-16,
-1.));
#12134=DIRECTION('ref_axis',(0.306109702391974,-0.9519962447938,-2.22431050430872E-16));
#12135=DIRECTION('center_axis',(-1.69724645484627E-17,-2.39104395366563E-16,
1.));
#12136=DIRECTION('ref_axis',(0.306109702391974,-0.9519962447938,-2.22431050430872E-16));
#12137=DIRECTION('center_axis',(0.999949654089045,0.010034405174207,1.93708804363157E-17));
#12138=DIRECTION('ref_axis',(-0.010034405174207,0.999949654089045,2.3892204885188E-16));
#12139=DIRECTION('',(1.69724645484627E-17,2.39104395366563E-16,-1.));
#12140=DIRECTION('',(-0.010034405174207,0.999949654089045,2.3892204885188E-16));
#12141=DIRECTION('',(0.010034405174207,-0.999949654089045,-2.3892204885188E-16));
#12142=DIRECTION('center_axis',(1.69724645484627E-17,2.39104395366563E-16,
-1.));
#12143=DIRECTION('ref_axis',(0.306109702391976,-0.9519962447938,-2.22431050430872E-16));
#12144=DIRECTION('',(1.69724645484627E-17,2.39104395366563E-16,-1.));
#12145=DIRECTION('center_axis',(1.69724645484627E-17,2.39104395366563E-16,
-1.));
#12146=DIRECTION('ref_axis',(0.306109702391976,-0.9519962447938,-2.22431050430872E-16));
#12147=DIRECTION('center_axis',(-1.69724645484627E-17,-2.39104395366563E-16,
1.));
#12148=DIRECTION('ref_axis',(0.306109702391976,-0.9519962447938,-2.22431050430872E-16));
#12149=DIRECTION('center_axis',(1.69724645484627E-17,2.39104395366563E-16,
-1.));
#12150=DIRECTION('ref_axis',(0.306109702391976,-0.9519962447938,-2.22431050430871E-16));
#12151=DIRECTION('center_axis',(-1.69724645484627E-17,-2.39104395366563E-16,
1.));
#12152=DIRECTION('ref_axis',(0.306109702391976,-0.9519962447938,-2.22431050430871E-16));
#12153=DIRECTION('center_axis',(1.69724645484627E-17,2.39104395366563E-16,
-1.));
#12154=DIRECTION('ref_axis',(0.306109702391976,-0.9519962447938,-2.22431050430871E-16));
#12155=DIRECTION('center_axis',(-0.306109702391976,0.9519962447938,2.22431050430871E-16));
#12156=DIRECTION('ref_axis',(-6.80883026501286E-17,2.1175352473573E-16,
-1.));
#12157=DIRECTION('center_axis',(-0.306109702391976,0.9519962447938,2.22431050430871E-16));
#12158=DIRECTION('ref_axis',(-6.80883026501286E-17,2.1175352473573E-16,
-1.));
#12159=DIRECTION('center_axis',(1.69724645484627E-17,2.39104395366563E-16,
-1.));
#12160=DIRECTION('ref_axis',(-0.310393882940736,0.950608035645067,0.));
#12161=DIRECTION('center_axis',(1.69724645484627E-17,2.39104395366563E-16,
-1.));
#12162=DIRECTION('ref_axis',(0.306109702391976,-0.9519962447938,0.));
#12163=DIRECTION('center_axis',(0.010034405174207,-0.999949654089045,-2.3892204885188E-16));
#12164=DIRECTION('ref_axis',(0.999949654089045,0.010034405174207,-2.9722020788518E-30));
#12165=DIRECTION('center_axis',(-0.306109702391976,0.9519962447938,2.22431050430871E-16));
#12166=DIRECTION('ref_axis',(-6.80883026501286E-17,2.1175352473573E-16,
-1.));
#12167=DIRECTION('center_axis',(1.69724645484627E-17,2.39104395366563E-16,
-1.));
#12168=DIRECTION('ref_axis',(0.306109702391976,-0.9519962447938,0.));
#12169=DIRECTION('center_axis',(0.873111609447877,-0.487520376443219,-1.0174940900013E-16));
#12170=DIRECTION('ref_axis',(0.487520376443219,0.873111609447877,1.56063105332704E-30));
#12171=DIRECTION('center_axis',(1.69724645484627E-17,2.39104395366563E-16,
-1.));
#12172=DIRECTION('ref_axis',(0.306109702391975,-0.9519962447938,0.));
#12173=DIRECTION('center_axis',(-0.010034405174207,0.999949654089045,2.3892204885188E-16));
#12174=DIRECTION('ref_axis',(-0.999949654089045,-0.010034405174207,2.9722020788518E-30));
#12175=DIRECTION('center_axis',(1.69724645484627E-17,2.39104395366563E-16,
-1.));
#12176=DIRECTION('ref_axis',(0.306109702391976,-0.9519962447938,0.));
#12177=DIRECTION('center_axis',(0.873111609447875,-0.487520376443223,-1.01749409000131E-16));
#12178=DIRECTION('ref_axis',(0.487520376443223,0.873111609447875,1.07581134523358E-30));
#12179=DIRECTION('center_axis',(1.69724645484627E-17,2.39104395366563E-16,
-1.));
#12180=DIRECTION('ref_axis',(-0.310393882940736,0.950608035645067,0.));
#12181=DIRECTION('center_axis',(0.306109702391976,-0.9519962447938,-2.22431050430871E-16));
#12182=DIRECTION('ref_axis',(6.80883026501286E-17,-2.1175352473573E-16,
1.));
#12183=DIRECTION('center_axis',(1.69724645484627E-17,2.39104395366563E-16,
-1.));
#12184=DIRECTION('ref_axis',(0.306109702391975,-0.9519962447938,0.));
#12185=DIRECTION('center_axis',(0.306109702391976,-0.9519962447938,-2.22431050430871E-16));
#12186=DIRECTION('ref_axis',(6.80883026501286E-17,-2.1175352473573E-16,
1.));
#12187=DIRECTION('center_axis',(1.69724645484627E-17,2.39104395366563E-16,
-1.));
#12188=DIRECTION('ref_axis',(0.306109702391976,-0.9519962447938,0.));
#12189=DIRECTION('center_axis',(0.306109702391976,-0.9519962447938,-2.22431050430871E-16));
#12190=DIRECTION('ref_axis',(6.80883026501286E-17,-2.1175352473573E-16,
1.));
#47413=CARTESIAN_POINT('',(0.,0.,0.));
#47414=CARTESIAN_POINT('Origin',(-70.1438101352762,-11.0431453779951,174.735485069079));
#47415=CARTESIAN_POINT('',(-70.7560295400602,-9.13915288840755,174.735485069079));
#47416=CARTESIAN_POINT('Origin',(-70.1438101352762,-11.0431453779951,174.735485069079));
#47417=CARTESIAN_POINT('',(-70.8325569656582,-8.9011538272091,174.485485069079));
#47418=CARTESIAN_POINT('Origin',(-70.8325569656582,-8.9011538272091,174.735485069079));
#47419=CARTESIAN_POINT('Origin',(-70.1438101352762,-11.0431453779951,174.485485069079));
#47420=CARTESIAN_POINT('Origin',(-53.6138862061095,-62.4509425968603,174.735485069079));
#47421=CARTESIAN_POINT('',(-57.8026696832023,-63.797825287385,174.735485069079));
#47422=CARTESIAN_POINT('',(-49.4251027290168,-61.1040599063356,174.735485069079));
#47423=CARTESIAN_POINT('Origin',(-53.6138862061095,-62.4509425968603,174.735485069079));
#47424=CARTESIAN_POINT('',(-57.5646706220038,-63.721297861787,174.485485069079));
#47425=CARTESIAN_POINT('Origin',(-57.5646706220038,-63.721297861787,174.735485069079));
#47426=CARTESIAN_POINT('',(-49.6631017902153,-61.1805873319336,174.485485069079));
#47427=CARTESIAN_POINT('Origin',(-53.6138862061095,-62.4509425968603,174.485485069079));
#47428=CARTESIAN_POINT('Origin',(-49.6631017902153,-61.1805873319336,174.735485069079));
#47429=CARTESIAN_POINT('Origin',(-53.6138862061095,-62.4509425968603,174.735485069079));
#47430=CARTESIAN_POINT('',(-54.2261056108935,-60.5469501072727,174.735485069079));
#47431=CARTESIAN_POINT('Origin',(-53.6138862061095,-62.4509425968603,174.735485069079));
#47432=CARTESIAN_POINT('',(-54.3026330364915,-60.3089510460743,174.485485069079));
#47433=CARTESIAN_POINT('Origin',(-54.3026330364915,-60.3089510460743,174.735485069079));
#47434=CARTESIAN_POINT('Origin',(-53.6138862061095,-62.4509425968603,174.485485069079));
#47435=CARTESIAN_POINT('Origin',(-53.6138862061095,-62.4509425968603,177.235485069079));
#47436=CARTESIAN_POINT('',(-57.5646706220038,-63.721297861787,177.485485069079));
#47437=CARTESIAN_POINT('',(-49.6631017902153,-61.1805873319336,177.485485069079));
#47438=CARTESIAN_POINT('Origin',(-53.6138862061095,-62.4509425968603,177.485485069079));
#47439=CARTESIAN_POINT('',(-57.8026696832023,-63.797825287385,177.235485069079));
#47440=CARTESIAN_POINT('Origin',(-57.5646706220038,-63.721297861787,177.235485069079));
#47441=CARTESIAN_POINT('',(-49.4251027290168,-61.1040599063356,177.235485069079));
#47442=CARTESIAN_POINT('Origin',(-53.6138862061095,-62.4509425968603,177.235485069079));
#47443=CARTESIAN_POINT('Origin',(-49.6631017902153,-61.1805873319336,177.235485069079));
#47444=CARTESIAN_POINT('Origin',(-70.1438101352762,-11.0431453779951,177.235485069079));
#47445=CARTESIAN_POINT('',(-70.8325569656582,-8.9011538272091,177.485485069079));
#47446=CARTESIAN_POINT('Origin',(-70.1438101352762,-11.0431453779951,177.485485069079));
#47447=CARTESIAN_POINT('',(-70.7560295400602,-9.13915288840755,177.235485069079));
#47448=CARTESIAN_POINT('Origin',(-70.8325569656582,-8.9011538272091,177.235485069079));
#47449=CARTESIAN_POINT('Origin',(-70.1438101352762,-11.0431453779951,177.235485069079));
#47450=CARTESIAN_POINT('Origin',(-53.6138862061095,-62.4509425968603,177.235485069079));
#47451=CARTESIAN_POINT('',(-54.3026330364915,-60.3089510460743,177.485485069079));
#47452=CARTESIAN_POINT('Origin',(-53.6138862061095,-62.4509425968603,177.485485069079));
#47453=CARTESIAN_POINT('',(-54.2261056108935,-60.5469501072727,177.235485069079));
#47454=CARTESIAN_POINT('Origin',(-54.3026330364915,-60.3089510460743,177.235485069079));
#47455=CARTESIAN_POINT('Origin',(-53.6138862061095,-62.4509425968603,177.235485069079));
#47456=CARTESIAN_POINT('Origin',(-53.6138862061095,-62.4509425968603,177.485485069079));
#47457=CARTESIAN_POINT('',(-54.2261056108935,-60.5469501072727,177.485485069079));
#47458=CARTESIAN_POINT('Origin',(-70.1438101352762,-11.0431453779951,177.485485069079));
#47459=CARTESIAN_POINT('',(-70.7560295400602,-9.13915288840755,177.485485069079));
#47460=CARTESIAN_POINT('Origin',(-53.6138862061095,-62.4509425968603,177.485485069079));
#47461=CARTESIAN_POINT('',(-57.8026696832023,-63.797825287385,177.485485069079));
#47462=CARTESIAN_POINT('',(-49.4251027290168,-61.1040599063356,177.485485069079));
#47463=CARTESIAN_POINT('Origin',(-53.6138862061095,-62.4509425968603,177.485485069079));
#47464=CARTESIAN_POINT('',(-73.7816789787941,-42.3755520783705,177.485485069079));
#47465=CARTESIAN_POINT('',(-68.8282104295052,-49.9715016156815,177.485485069079));
#47466=CARTESIAN_POINT('Origin',(-64.0748867591837,-41.4586634235648,177.485485069079));
#47467=CARTESIAN_POINT('Origin',(-80.6505795582534,-71.1444581447924,177.485485069079));
#47468=CARTESIAN_POINT('',(-54.8465294930114,-45.0602106510818,177.485485069079));
#47469=CARTESIAN_POINT('',(-49.6631017902153,-61.1805873319336,177.485485069079));
#47470=CARTESIAN_POINT('',(-61.0095980165858,-25.8931667939203,177.485485069079));
#47471=CARTESIAN_POINT('Origin',(-41.2010060476238,-30.0981857245761,177.485485069079));
#47472=CARTESIAN_POINT('',(-66.193025719382,-9.77279011306845,177.485485069079));
#47473=CARTESIAN_POINT('',(-49.6631017902153,-61.1805873319336,177.485485069079));
#47474=CARTESIAN_POINT('',(-74.082992404925,-12.3490332163964,177.485485069079));
#47475=CARTESIAN_POINT('Origin',(-70.1438101352762,-11.0431453779951,177.485485069079));
#47476=CARTESIAN_POINT('',(-73.5782138375345,-62.6512828356565,177.485485069079));
#47477=CARTESIAN_POINT('Origin',(-53.6138862061095,-62.4509425968603,174.485485069079));
#47478=CARTESIAN_POINT('',(-61.0095980165858,-25.8931667939203,174.485485069079));
#47479=CARTESIAN_POINT('',(-54.8465294930114,-45.0602106510818,174.485485069079));
#47480=CARTESIAN_POINT('Origin',(-41.2010060476238,-30.0981857245761,174.485485069079));
#47481=CARTESIAN_POINT('',(-49.6631017902153,-61.1805873319336,174.485485069079));
#47482=CARTESIAN_POINT('',(-68.8282104295052,-49.9715016156815,174.485485069079));
#47483=CARTESIAN_POINT('Origin',(-80.6505795582534,-71.1444581447924,174.485485069079));
#47484=CARTESIAN_POINT('',(-73.7816789787941,-42.3755520783705,174.485485069079));
#47485=CARTESIAN_POINT('Origin',(-64.0748867591837,-41.4586634235648,174.485485069079));
#47486=CARTESIAN_POINT('',(-74.082992404925,-12.3490332163964,174.485485069079));
#47487=CARTESIAN_POINT('',(-74.0826061988467,-12.3875194672263,174.485485069079));
#47488=CARTESIAN_POINT('',(-66.193025719382,-9.77279011306845,174.485485069079));
#47489=CARTESIAN_POINT('Origin',(-70.1438101352762,-11.0431453779951,174.485485069079));
#47490=CARTESIAN_POINT('',(-60.9891607787184,-25.956726274563,174.485485069079));
#47491=CARTESIAN_POINT('Origin',(-49.4251027290168,-61.1040599063356,177.485485069079));
#47492=CARTESIAN_POINT('',(-54.6289676696804,-44.920123744841,177.235485069079));
#47493=CARTESIAN_POINT('',(-54.6289676696804,-44.920123744841,174.735485069079));
#47494=CARTESIAN_POINT('',(-54.6289676696804,-44.920123744841,177.485485069079));
#47495=CARTESIAN_POINT('',(-49.4251027290168,-61.1040599063356,177.235485069079));
#47496=CARTESIAN_POINT('',(-54.6289676696804,-44.920123744841,174.735485069079));
#47497=CARTESIAN_POINT('Origin',(-41.2010060476238,-30.0981857245761,177.485485069079));
#47498=CARTESIAN_POINT('',(-60.7511617175199,-25.8801988489651,177.235485069079));
#47499=CARTESIAN_POINT('',(-60.7511617175199,-25.8801988489651,174.735485069079));
#47500=CARTESIAN_POINT('',(-60.7511617175199,-25.8801988489651,177.485485069079));
#47501=CARTESIAN_POINT('Origin',(-41.2010060476238,-30.0981857245761,177.235485069079));
#47502=CARTESIAN_POINT('Origin',(-41.2010060476238,-30.0981857245761,174.735485069079));
#47503=CARTESIAN_POINT('Origin',(-60.7511617175199,-25.8801988489651,177.485485069079));
#47504=CARTESIAN_POINT('',(-65.9550266581835,-9.69626268747045,177.235485069079));
#47505=CARTESIAN_POINT('',(-65.9550266581835,-9.69626268747045,174.735485069079));
#47506=CARTESIAN_POINT('',(-65.9550266581835,-9.69626268747045,177.485485069079));
#47507=CARTESIAN_POINT('',(-60.7511617175199,-25.8801988489651,177.235485069079));
#47508=CARTESIAN_POINT('',(-65.9550266581835,-9.69626268747045,174.735485069079));
#47509=CARTESIAN_POINT('Origin',(-70.1438101352762,-11.0431453779951,177.485485069079));
#47510=CARTESIAN_POINT('',(-74.3325936123689,-12.3900280685198,177.235485069079));
#47511=CARTESIAN_POINT('',(-74.3325936123689,-12.3900280685198,174.735485069079));
#47512=CARTESIAN_POINT('',(-74.3325936123689,-12.3900280685198,177.485485069079));
#47513=CARTESIAN_POINT('Origin',(-70.1438101352762,-11.0431453779951,177.235485069079));
#47514=CARTESIAN_POINT('Origin',(-70.1438101352762,-11.0431453779951,174.735485069079));
#47515=CARTESIAN_POINT('Origin',(-74.0315614571427,-42.3885176911912,177.485485069079));
#47516=CARTESIAN_POINT('',(-74.0315614571427,-42.3885176911912,177.235485069079));
#47517=CARTESIAN_POINT('',(-74.0315614571427,-42.3885176911912,174.735485069079));
#47518=CARTESIAN_POINT('',(-74.0315614571427,-42.3885176911912,177.485485069079));
#47519=CARTESIAN_POINT('',(-74.0315614571427,-42.3885176911912,177.235485069079));
#47520=CARTESIAN_POINT('',(-74.0315614571427,-42.3885176911912,174.735485069079));
#47521=CARTESIAN_POINT('Origin',(-64.0748867591837,-41.4586634235648,177.485485069079));
#47522=CARTESIAN_POINT('',(-68.950090523616,-50.1897795180435,177.235485069079));
#47523=CARTESIAN_POINT('',(-68.950090523616,-50.1897795180435,174.735485069079));
#47524=CARTESIAN_POINT('',(-68.950090523616,-50.1897795180435,177.485485069079));
#47525=CARTESIAN_POINT('Origin',(-64.0748867591837,-41.4586634235648,177.235485069079));
#47526=CARTESIAN_POINT('Origin',(-64.0748867591837,-41.4586634235648,174.735485069079));
#47527=CARTESIAN_POINT('Origin',(-80.6505795582534,-71.1444581447924,177.485485069079));
#47528=CARTESIAN_POINT('Origin',(-80.6505795582534,-71.1444581447924,177.235485069079));
#47529=CARTESIAN_POINT('Origin',(-80.6505795582534,-71.1444581447924,174.735485069079));
#47530=CARTESIAN_POINT('Origin',(-49.6631017902153,-61.1805873319336,177.235485069079));
#47531=CARTESIAN_POINT('Ctrl Pts',(-60.7511617175199,-25.8801988489651,
177.235485069079));
#47532=CARTESIAN_POINT('Ctrl Pts',(-60.7511617175199,-25.8801988489651,
177.236209624631));
#47533=CARTESIAN_POINT('Ctrl Pts',(-60.7511649745547,-25.8801990096816,
177.236934363604));
#47534=CARTESIAN_POINT('Ctrl Pts',(-60.751454897117,-25.8802133157759,177.26917313906));
#47535=CARTESIAN_POINT('Ctrl Pts',(-60.7578951724417,-25.8805307741899,
177.300270548243));
#47536=CARTESIAN_POINT('Ctrl Pts',(-60.782469053451,-25.8817463747679,177.358946342665));
#47537=CARTESIAN_POINT('Ctrl Pts',(-60.8005420012037,-25.8826417492884,
177.385802945446));
#47538=CARTESIAN_POINT('Ctrl Pts',(-60.8465753700736,-25.8849347071446,
177.432198391808));
#47539=CARTESIAN_POINT('Ctrl Pts',(-60.8744154272029,-25.88632691736,177.450986825543));
#47540=CARTESIAN_POINT('Ctrl Pts',(-60.937307891463,-25.8894927969754,177.477924595734));
#47541=CARTESIAN_POINT('Ctrl Pts',(-60.9721283554826,-25.8912560982159,
177.48517070955));
#47542=CARTESIAN_POINT('Ctrl Pts',(-61.0080570542599,-25.8930881990745,
177.48548173422));
#47543=CARTESIAN_POINT('Ctrl Pts',(-61.0088275341472,-25.8931274935949,
177.485485069079));
#47544=CARTESIAN_POINT('Ctrl Pts',(-61.0095980165858,-25.8931667939203,
177.485485069079));
#47545=CARTESIAN_POINT('Origin',(-66.193025719382,-9.77279011306845,177.235485069079));
#47546=CARTESIAN_POINT('Origin',(-70.1438101352762,-11.0431453779951,177.235485069079));
#47547=CARTESIAN_POINT('Ctrl Pts',(-74.0829924049255,-12.3490332163965,
177.485485069079));
#47548=CARTESIAN_POINT('Ctrl Pts',(-74.0837490876437,-12.3491592710996,
177.485485069079));
#47549=CARTESIAN_POINT('Ctrl Pts',(-74.0845057695073,-12.3492853090228,
177.485481622518));
#47550=CARTESIAN_POINT('Ctrl Pts',(-74.1187223288458,-12.3549838920991,
177.485169912202));
#47551=CARTESIAN_POINT('Ctrl Pts',(-74.1518167082703,-12.3604619039869,
177.478128415433));
#47552=CARTESIAN_POINT('Ctrl Pts',(-74.2122917073814,-12.3704217394355,
177.451777056831));
#47553=CARTESIAN_POINT('Ctrl Pts',(-74.2392789041521,-12.3748411885359,
177.433118690759));
#47554=CARTESIAN_POINT('Ctrl Pts',(-74.2843931866928,-12.3822052137679,
177.386633798983));
#47555=CARTESIAN_POINT('Ctrl Pts',(-74.3021911232899,-12.3850970696903,
177.359357331601));
#47556=CARTESIAN_POINT('Ctrl Pts',(-74.3263794660467,-12.3890225555062,
177.29957394136));
#47557=CARTESIAN_POINT('Ctrl Pts',(-74.332593612369,-12.3900280685198,177.267693581309));
#47558=CARTESIAN_POINT('Ctrl Pts',(-74.3325936123689,-12.3900280685198,
177.235485069079));
#47559=CARTESIAN_POINT('Origin',(-41.2010060476238,-30.0981857245761,177.235485069079));
#47560=CARTESIAN_POINT('Ctrl Pts',(-54.6289676696804,-44.920123744841,177.235485069079));
#47561=CARTESIAN_POINT('Ctrl Pts',(-54.6289676696804,-44.9201237448411,
177.266555445342));
#47562=CARTESIAN_POINT('Ctrl Pts',(-54.6340056002196,-44.9233739545679,
177.297288535147));
#47563=CARTESIAN_POINT('Ctrl Pts',(-54.6540860524352,-44.9363240585933,
177.356614103802));
#47564=CARTESIAN_POINT('Ctrl Pts',(-54.6694432684634,-44.9462265480297,
177.384289371841));
#47565=CARTESIAN_POINT('Ctrl Pts',(-54.7089373275903,-44.9716773681615,
177.432038662699));
#47566=CARTESIAN_POINT('Ctrl Pts',(-54.7329702784393,-44.9871579385665,
177.451300874194));
#47567=CARTESIAN_POINT('Ctrl Pts',(-54.7863463486712,-45.0215139393215,
177.478097428015));
#47568=CARTESIAN_POINT('Ctrl Pts',(-54.8153235492639,-45.0401531604041,
177.485174360859));
#47569=CARTESIAN_POINT('Ctrl Pts',(-54.845231509254,-45.0593763968009,177.48548173422));
#47570=CARTESIAN_POINT('Ctrl Pts',(-54.8458804984045,-45.0597935255564,
177.485485069079));
#47571=CARTESIAN_POINT('Ctrl Pts',(-54.8465294930115,-45.0602106510817,
177.485485069079));
#47572=CARTESIAN_POINT('Origin',(-73.5782138375345,-62.6512828356565,177.235485069079));
#47573=CARTESIAN_POINT('Ctrl Pts',(-73.7816789787941,-42.3755520783705,
177.485485069079));
#47574=CARTESIAN_POINT('Ctrl Pts',(-73.7981057833924,-42.3764086084212,
177.485485069079));
#47575=CARTESIAN_POINT('Ctrl Pts',(-73.8145162527323,-42.3772651018765,
177.483859254794));
#47576=CARTESIAN_POINT('Ctrl Pts',(-73.8305939553847,-42.3781032802876,
177.48064835975));
#47577=CARTESIAN_POINT('Ctrl Pts',(-73.8459401365431,-42.3789033223096,
177.47758355764));
#47578=CARTESIAN_POINT('Ctrl Pts',(-73.8609825651133,-42.379686630563,177.473075252585));
#47579=CARTESIAN_POINT('Ctrl Pts',(-73.8754594678907,-42.38043896216,177.467210817261));
#47580=CARTESIAN_POINT('Ctrl Pts',(-73.889953215135,-42.3811921691254,177.461339558427));
#47581=CARTESIAN_POINT('Ctrl Pts',(-73.9038795299571,-42.3819142779909,
177.45410931481));
#47582=CARTESIAN_POINT('Ctrl Pts',(-73.9169982217908,-42.3825934214874,
177.445654854873));
#47583=CARTESIAN_POINT('Ctrl Pts',(-73.9301452183313,-42.3832740302944,
177.43718215371));
#47584=CARTESIAN_POINT('Ctrl Pts',(-73.9424805770332,-42.3839114468893,
177.427480351751));
#47585=CARTESIAN_POINT('Ctrl Pts',(-73.9537935453965,-42.3844968441549,
177.416727042628));
#47586=CARTESIAN_POINT('Ctrl Pts',(-73.9553553902192,-42.3845776628807,
177.415242463193));
#47587=CARTESIAN_POINT('Ctrl Pts',(-73.9568978035099,-42.3846574955071,
177.4137379014));
#47588=CARTESIAN_POINT('Ctrl Pts',(-73.9584202852857,-42.3847363240965,
177.412213879973));
#47589=CARTESIAN_POINT('Ctrl Pts',(-73.9702299481194,-42.3853477856444,
177.400392274298));
#47590=CARTESIAN_POINT('Ctrl Pts',(-73.9808446692677,-42.3858989380282,
177.387389529667));
#47591=CARTESIAN_POINT('Ctrl Pts',(-73.9900643178673,-42.3863772577204,
177.373450709894));
#47592=CARTESIAN_POINT('Ctrl Pts',(-73.9992576720282,-42.3868542132448,
177.359551643636));
#47593=CARTESIAN_POINT('Ctrl Pts',(-74.0070636659419,-42.3872587376246,
177.344722141989));
#47594=CARTESIAN_POINT('Ctrl Pts',(-74.0133253949135,-42.3875821461516,
177.329235611602));
#47595=CARTESIAN_POINT('Ctrl Pts',(-74.0195252880819,-42.3879023609559,
177.313902013744));
#47596=CARTESIAN_POINT('Ctrl Pts',(-74.0242110678826,-42.3881430426806,
177.297924635572));
#47597=CARTESIAN_POINT('Ctrl Pts',(-74.0272743187926,-42.3882996010354,
177.281593926282));
#47598=CARTESIAN_POINT('Ctrl Pts',(-74.0301158269513,-42.3884448264367,
177.266445365145));
#47599=CARTESIAN_POINT('Ctrl Pts',(-74.0315614571427,-42.3885176911912,
177.250993231542));
#47600=CARTESIAN_POINT('Ctrl Pts',(-74.0315614571427,-42.3885176911912,
177.235485069079));
#47601=CARTESIAN_POINT('Origin',(-49.6631017902153,-61.1805873319336,177.235485069079));
#47602=CARTESIAN_POINT('Origin',(-64.0748867591837,-41.4586634235648,177.235485069079));
#47603=CARTESIAN_POINT('Origin',(-68.8282104295052,-49.9715016156815,177.235485069079));
#47604=CARTESIAN_POINT('Origin',(-80.6505795582534,-71.1444581447924,177.235485069079));
#47605=CARTESIAN_POINT('Origin',(-73.7815740436205,-42.3860090898976,174.735485069079));
#47606=CARTESIAN_POINT('Ctrl Pts',(-74.0829924049252,-12.3490332163965,
174.485485069079));
#47607=CARTESIAN_POINT('Ctrl Pts',(-74.0837490876434,-12.3491592710996,
174.485485069079));
#47608=CARTESIAN_POINT('Ctrl Pts',(-74.0845057695072,-12.3492853090228,
174.48548851564));
#47609=CARTESIAN_POINT('Ctrl Pts',(-74.1187223288457,-12.3549838920989,
174.485800225956));
#47610=CARTESIAN_POINT('Ctrl Pts',(-74.1518167082703,-12.3604619039867,
174.492841722725));
#47611=CARTESIAN_POINT('Ctrl Pts',(-74.2122917073815,-12.3704217394354,
174.519193081327));
#47612=CARTESIAN_POINT('Ctrl Pts',(-74.2392789041521,-12.374841188536,174.5378514474));
#47613=CARTESIAN_POINT('Ctrl Pts',(-74.2843931866929,-12.3822052137679,
174.584336339176));
#47614=CARTESIAN_POINT('Ctrl Pts',(-74.3021911232899,-12.3850970696904,
174.611612806557));
#47615=CARTESIAN_POINT('Ctrl Pts',(-74.3263794660467,-12.3890225555062,
174.671396196798));
#47616=CARTESIAN_POINT('Ctrl Pts',(-74.3325936123689,-12.3900280685199,
174.70327655685));
#47617=CARTESIAN_POINT('Ctrl Pts',(-74.3325936123689,-12.3900280685199,
174.735485069079));
#47618=CARTESIAN_POINT('Ctrl Pts',(-74.0315614571427,-42.3885176911912,
174.735485069079));
#47619=CARTESIAN_POINT('Ctrl Pts',(-74.0315614571427,-42.3885176911912,
174.718765393872));
#47620=CARTESIAN_POINT('Ctrl Pts',(-74.0298805568919,-42.3884329506508,
174.702110999624));
#47621=CARTESIAN_POINT('Ctrl Pts',(-74.026582879632,-42.3882642507143,174.685831471344));
#47622=CARTESIAN_POINT('Ctrl Pts',(-74.02326312362,-42.3880944212906,174.669442947658));
#47623=CARTESIAN_POINT('Ctrl Pts',(-74.0183051173532,-42.3878395216834,
174.653434683319));
#47624=CARTESIAN_POINT('Ctrl Pts',(-74.0118230397663,-42.3875045410618,
174.638101343067));
#47625=CARTESIAN_POINT('Ctrl Pts',(-74.0053026648678,-42.3871675813129,
174.62267741061));
#47626=CARTESIAN_POINT('Ctrl Pts',(-73.9972403916431,-42.3867496058168,
174.607936732203));
#47627=CARTESIAN_POINT('Ctrl Pts',(-73.9877979397281,-42.3862596813854,
174.594152694406));
#47628=CARTESIAN_POINT('Ctrl Pts',(-73.9791080850659,-42.3858088056868,
174.581467293813));
#47629=CARTESIAN_POINT('Ctrl Pts',(-73.9692499366581,-42.3852970451061,
174.569592003359));
#47630=CARTESIAN_POINT('Ctrl Pts',(-73.9583807640474,-42.3847342778285,
174.558716705829));
#47631=CARTESIAN_POINT('Ctrl Pts',(-73.9481748997668,-42.384205854308,174.548505090413));
#47632=CARTESIAN_POINT('Ctrl Pts',(-73.937051290793,-42.3836314002962,174.539151069091));
#47633=CARTESIAN_POINT('Ctrl Pts',(-73.9251817152964,-42.3830174841342,
174.530820820265));
#47634=CARTESIAN_POINT('Ctrl Pts',(-73.91332102571,-42.3824040275676,174.522496807706));
#47635=CARTESIAN_POINT('Ctrl Pts',(-73.9007161293092,-42.3817512215404,
174.515195584145));
#47636=CARTESIAN_POINT('Ctrl Pts',(-73.8875713433795,-42.3810688619176,
174.509042800644));
#47637=CARTESIAN_POINT('Ctrl Pts',(-73.8744327327308,-42.3803868228602,
174.502892907656));
#47638=CARTESIAN_POINT('Ctrl Pts',(-73.8607555029461,-42.3796753245276,
174.497890739208));
#47639=CARTESIAN_POINT('Ctrl Pts',(-73.8467659990825,-42.3789464847267,
174.494114765878));
#47640=CARTESIAN_POINT('Ctrl Pts',(-73.8327506058318,-42.3782162961134,
174.490331804621));
#47641=CARTESIAN_POINT('Ctrl Pts',(-73.8184226118037,-42.3774687767553,
174.487779751606));
#47642=CARTESIAN_POINT('Ctrl Pts',(-73.8040200140351,-42.3767173904492,
174.486486267331));
#47643=CARTESIAN_POINT('Ctrl Pts',(-73.796581894898,-42.3763293423378,174.485818256581));
#47644=CARTESIAN_POINT('Ctrl Pts',(-73.7891239696738,-42.375940276719,174.485485069079));
#47645=CARTESIAN_POINT('Ctrl Pts',(-73.7816789787941,-42.3755520783705,
174.485485069079));
#47646=CARTESIAN_POINT('Origin',(-64.0748867591837,-41.4586634235648,174.735485069079));
#47647=CARTESIAN_POINT('Origin',(-68.8282104295052,-49.9715016156815,174.735485069079));
#47648=CARTESIAN_POINT('Origin',(-70.1438101352762,-11.0431453779951,174.735485069079));
#47649=CARTESIAN_POINT('Origin',(-66.193025719382,-9.77279011306845,174.735485069079));
#47650=CARTESIAN_POINT('Origin',(-80.6505795582534,-71.1444581447924,174.735485069079));
#47651=CARTESIAN_POINT('Origin',(-60.9891607787184,-25.956726274563,174.735485069079));
#47652=CARTESIAN_POINT('Ctrl Pts',(-61.0095980165858,-25.8931667939203,
174.485485069079));
#47653=CARTESIAN_POINT('Ctrl Pts',(-61.0088275341472,-25.8931274935949,
174.485485069079));
#47654=CARTESIAN_POINT('Ctrl Pts',(-61.0080570542599,-25.8930881990744,
174.485488403939));
#47655=CARTESIAN_POINT('Ctrl Pts',(-60.9725501444756,-25.8912776063701,
174.4857957773));
#47656=CARTESIAN_POINT('Ctrl Pts',(-60.9381399458952,-25.8895349215335,
174.492872710144));
#47657=CARTESIAN_POINT('Ctrl Pts',(-60.8747431598305,-25.8863431856417,
174.519669263965));
#47658=CARTESIAN_POINT('Ctrl Pts',(-60.8461915856332,-25.8849154610819,
174.53893147546));
#47659=CARTESIAN_POINT('Ctrl Pts',(-60.7992654458767,-25.8825782920219,
174.586680766318));
#47660=CARTESIAN_POINT('Ctrl Pts',(-60.781014795274,-25.8816743375162,174.614356034357));
#47661=CARTESIAN_POINT('Ctrl Pts',(-60.7571498297398,-25.8804940089663,
174.673681603012));
#47662=CARTESIAN_POINT('Ctrl Pts',(-60.7511617175199,-25.8801988489651,
174.704414692817));
#47663=CARTESIAN_POINT('Ctrl Pts',(-60.7511617175199,-25.8801988489651,
174.735485069079));
#47664=CARTESIAN_POINT('Origin',(-41.2010060476238,-30.0981857245761,174.735485069079));
#47665=CARTESIAN_POINT('Ctrl Pts',(-54.8465294930115,-45.0602106510817,
174.485485069079));
#47666=CARTESIAN_POINT('Ctrl Pts',(-54.8458804984045,-45.0597935255564,
174.485485069079));
#47667=CARTESIAN_POINT('Ctrl Pts',(-54.845231509254,-45.0593763968009,174.485488403939));
#47668=CARTESIAN_POINT('Ctrl Pts',(-54.8153235492641,-45.0401531604042,
174.4857957773));
#47669=CARTESIAN_POINT('Ctrl Pts',(-54.7863463486712,-45.0215139393217,
174.492872710144));
#47670=CARTESIAN_POINT('Ctrl Pts',(-54.7329702784391,-44.9871579385665,
174.519669263965));
#47671=CARTESIAN_POINT('Ctrl Pts',(-54.7089373275902,-44.9716773681615,
174.538931475459));
#47672=CARTESIAN_POINT('Ctrl Pts',(-54.6694432684634,-44.9462265480297,
174.586680766317));
#47673=CARTESIAN_POINT('Ctrl Pts',(-54.6540860524352,-44.9363240585933,
174.614356034356));
#47674=CARTESIAN_POINT('Ctrl Pts',(-54.6340056002196,-44.9233739545679,
174.673681603011));
#47675=CARTESIAN_POINT('Ctrl Pts',(-54.6289676696804,-44.920123744841,174.704414692817));
#47676=CARTESIAN_POINT('Ctrl Pts',(-54.6289676696804,-44.920123744841,174.735485069079));
#47677=CARTESIAN_POINT('Origin',(-49.6631017902153,-61.1805873319336,174.735485069079));
#47702=UNCERTAINTY_MEASURE_WITH_UNIT(LENGTH_MEASURE(0.01),#47718,
'DISTANCE_ACCURACY_VALUE',
'Maximum model space distance between geometric entities at asserted c
onnectivities');
#47703=UNCERTAINTY_MEASURE_WITH_UNIT(LENGTH_MEASURE(0.01),#47718,
'DISTANCE_ACCURACY_VALUE',
'Maximum model space distance between geometric entities at asserted c
onnectivities');
#47716=(
GEOMETRIC_REPRESENTATION_CONTEXT(3)
GLOBAL_UNCERTAINTY_ASSIGNED_CONTEXT((#47702))
GLOBAL_UNIT_ASSIGNED_CONTEXT((#47718,#47720,#47721))
REPRESENTATION_CONTEXT('','3D')
);
#47717=(
GEOMETRIC_REPRESENTATION_CONTEXT(3)
GLOBAL_UNCERTAINTY_ASSIGNED_CONTEXT((#47703))
GLOBAL_UNIT_ASSIGNED_CONTEXT((#47718,#47720,#47721))
REPRESENTATION_CONTEXT('','3D')
);
#47718=(
LENGTH_UNIT()
NAMED_UNIT(*)
SI_UNIT(.MILLI.,.METRE.)
);
#47720=(
NAMED_UNIT(*)
PLANE_ANGLE_UNIT()
SI_UNIT($,.RADIAN.)
);
#47721=(
NAMED_UNIT(*)
SI_UNIT($,.STERADIAN.)
SOLID_ANGLE_UNIT()
);
#47734=SHAPE_DEFINITION_REPRESENTATION(#47747,#47772);
#47747=PRODUCT_DEFINITION_SHAPE('',$,#47786);
#47772=SHAPE_REPRESENTATION('',(#9871),#47716);
#47773=PRODUCT_DEFINITION_CONTEXT('part definition',#47814,'design');
#47786=PRODUCT_DEFINITION('Link Lever','Link Lever',#47799,#47773);
#47799=PRODUCT_DEFINITION_FORMATION('',$,#47828);
#47814=APPLICATION_CONTEXT(
'Core Data for Automotive Mechanical Design Process');
#47815=PRODUCT_CONTEXT('part definition',#47814,'mechanical');
#47828=PRODUCT('Link Lever','Link Lever',$,(#47815));
#47830=PRESENTATION_STYLE_ASSIGNMENT((#47832));
#47832=SURFACE_STYLE_USAGE(.BOTH.,#47834);
#47834=SURFACE_SIDE_STYLE('',(#47836));
#47836=SURFACE_STYLE_FILL_AREA(#47838);
#47838=FILL_AREA_STYLE('Opaque(202,209,238)',(#47840));
#47840=FILL_AREA_STYLE_COLOUR('Opaque(202,209,238)',#47842);
#47842=COLOUR_RGB('Opaque(202,209,238)', 0.66274510, 0.83137255, 0.94901961);
ENDSEC;
END-ISO-10303-21;
